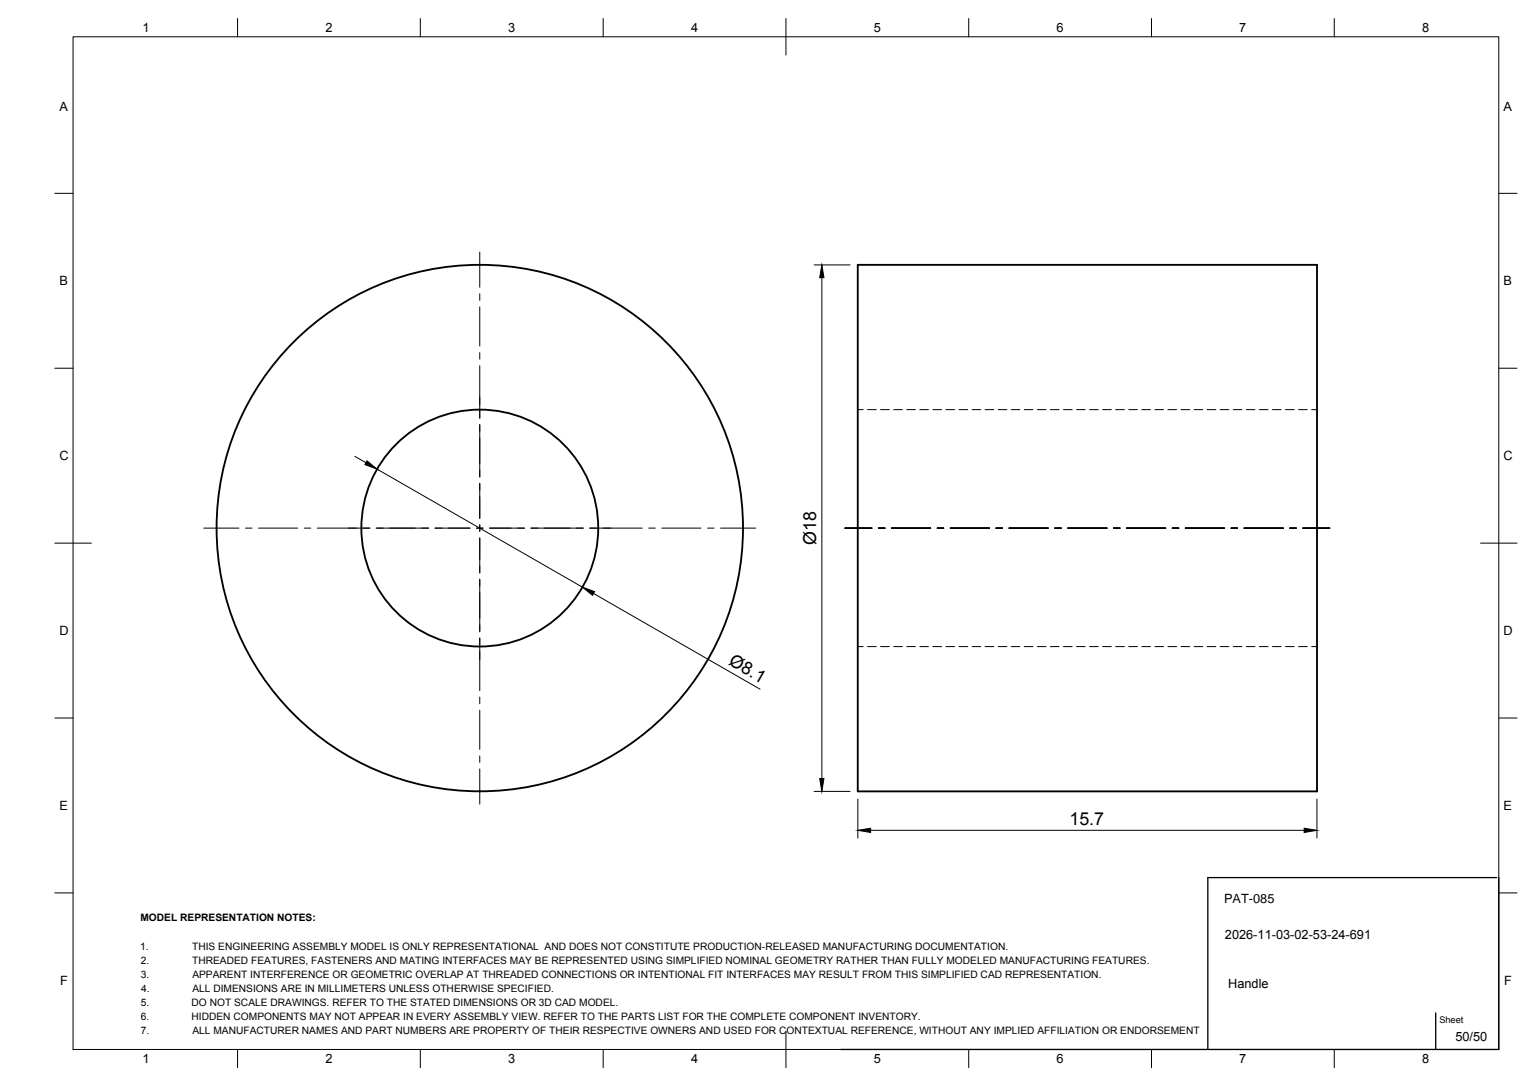
ISO-10303-21;
HEADER;
/* Generated by software containing ST-Developer
 * from STEP Tools, Inc. (www.steptools.com) 
 */

FILE_DESCRIPTION(
/* description */ ('Rack and pinion manual slide'),
/* implementation_level */ '2;1');

FILE_NAME(
/* name */ 'Handle.step',
/* time_stamp */ '2026-10-28T03:22:49-07:00',
/* author */ (''),
/* organization */ (''),
/* preprocessor_version */ 'ST-DEVELOPER v20.2',
/* originating_system */ 'Autodesk Translation Framework v15.17.0.0',
/* authorisation */ '');

FILE_SCHEMA (('AUTOMOTIVE_DESIGN { 1 0 10303 214 3 1 1 }'));
ENDSEC;

DATA;
#10=MECHANICAL_DESIGN_GEOMETRIC_PRESENTATION_REPRESENTATION('',(#784),#34851);
#685=SHAPE_REPRESENTATION_RELATIONSHIP('SRR','None',#35125,#731);
#731=ADVANCED_BREP_SHAPE_REPRESENTATION('',(#832),#34850);
#784=STYLED_ITEM('',(#35404),#832);
#832=MANIFOLD_SOLID_BREP('Body1',#13809);
#1042=FACE_BOUND('',#3221,.T.);
#1043=FACE_BOUND('',#3223,.T.);
#1533=PLANE('',#15593);
#1534=PLANE('',#15594);
#2270=FACE_OUTER_BOUND('',#3218,.T.);
#2271=FACE_OUTER_BOUND('',#3219,.T.);
#2272=FACE_OUTER_BOUND('',#3220,.T.);
#2273=FACE_OUTER_BOUND('',#3222,.T.);
#3218=EDGE_LOOP('',(#12832,#12833,#12834,#12835));
#3219=EDGE_LOOP('',(#12836,#12837,#12838,#12839));
#3220=EDGE_LOOP('',(#12840));
#3221=EDGE_LOOP('',(#12841));
#3222=EDGE_LOOP('',(#12842));
#3223=EDGE_LOOP('',(#12843));
#4513=LINE('',#34729,#5804);
#4514=LINE('',#34735,#5805);
#5804=VECTOR('',#19433,0.404999999999999);
#5805=VECTOR('',#19440,0.9);
#6220=CIRCLE('',#15588,0.404999999999999);
#6221=CIRCLE('',#15589,0.404999999999999);
#6222=CIRCLE('',#15591,0.9);
#6223=CIRCLE('',#15592,0.9);
#7425=VERTEX_POINT('',#34726);
#7426=VERTEX_POINT('',#34728);
#7427=VERTEX_POINT('',#34732);
#7428=VERTEX_POINT('',#34734);
#9228=EDGE_CURVE('',#7425,#7425,#6220,.T.);
#9229=EDGE_CURVE('',#7425,#7426,#4513,.T.);
#9230=EDGE_CURVE('',#7426,#7426,#6221,.T.);
#9231=EDGE_CURVE('',#7427,#7427,#6222,.T.);
#9232=EDGE_CURVE('',#7427,#7428,#4514,.T.);
#9233=EDGE_CURVE('',#7428,#7428,#6223,.T.);
#12832=ORIENTED_EDGE('',*,*,#9228,.F.);
#12833=ORIENTED_EDGE('',*,*,#9229,.T.);
#12834=ORIENTED_EDGE('',*,*,#9230,.T.);
#12835=ORIENTED_EDGE('',*,*,#9229,.F.);
#12836=ORIENTED_EDGE('',*,*,#9231,.F.);
#12837=ORIENTED_EDGE('',*,*,#9232,.T.);
#12838=ORIENTED_EDGE('',*,*,#9233,.T.);
#12839=ORIENTED_EDGE('',*,*,#9232,.F.);
#12840=ORIENTED_EDGE('',*,*,#9231,.T.);
#12841=ORIENTED_EDGE('',*,*,#9228,.T.);
#12842=ORIENTED_EDGE('',*,*,#9233,.F.);
#12843=ORIENTED_EDGE('',*,*,#9230,.F.);
#13011=CYLINDRICAL_SURFACE('',#15587,0.404999999999999);
#13012=CYLINDRICAL_SURFACE('',#15590,0.9);
#13748=ADVANCED_FACE('',(#2270),#13011,.F.);
#13749=ADVANCED_FACE('',(#2271),#13012,.T.);
#13750=ADVANCED_FACE('',(#2272,#1042),#1533,.T.);
#13751=ADVANCED_FACE('',(#2273,#1043),#1534,.F.);
#13809=CLOSED_SHELL('',(#13748,#13749,#13750,#13751));
#15586=AXIS2_PLACEMENT_3D('',#34724,#19427,#19428);
#15587=AXIS2_PLACEMENT_3D('',#34725,#19429,#19430);
#15588=AXIS2_PLACEMENT_3D('',#34727,#19431,#19432);
#15589=AXIS2_PLACEMENT_3D('',#34730,#19434,#19435);
#15590=AXIS2_PLACEMENT_3D('',#34731,#19436,#19437);
#15591=AXIS2_PLACEMENT_3D('',#34733,#19438,#19439);
#15592=AXIS2_PLACEMENT_3D('',#34736,#19441,#19442);
#15593=AXIS2_PLACEMENT_3D('',#34737,#19443,#19444);
#15594=AXIS2_PLACEMENT_3D('',#34738,#19445,#19446);
#19427=DIRECTION('axis',(0.,0.,1.));
#19428=DIRECTION('refdir',(1.,0.,0.));
#19429=DIRECTION('center_axis',(0.,1.,0.));
#19430=DIRECTION('ref_axis',(1.,0.,0.));
#19431=DIRECTION('center_axis',(0.,-1.,0.));
#19432=DIRECTION('ref_axis',(1.,0.,0.));
#19433=DIRECTION('',(0.,-1.,0.));
#19434=DIRECTION('center_axis',(0.,-1.,0.));
#19435=DIRECTION('ref_axis',(1.,0.,0.));
#19436=DIRECTION('center_axis',(0.,1.,0.));
#19437=DIRECTION('ref_axis',(1.,0.,0.));
#19438=DIRECTION('center_axis',(0.,1.,0.));
#19439=DIRECTION('ref_axis',(1.,0.,0.));
#19440=DIRECTION('',(0.,-1.,0.));
#19441=DIRECTION('center_axis',(0.,1.,0.));
#19442=DIRECTION('ref_axis',(1.,0.,0.));
#19443=DIRECTION('center_axis',(0.,1.,0.));
#19444=DIRECTION('ref_axis',(1.,0.,0.));
#19445=DIRECTION('center_axis',(0.,1.,0.));
#19446=DIRECTION('ref_axis',(1.,0.,0.));
#34724=CARTESIAN_POINT('',(0.,0.,0.));
#34725=CARTESIAN_POINT('Origin',(11.,7.3,13.25));
#34726=CARTESIAN_POINT('',(10.595,8.87,13.25));
#34727=CARTESIAN_POINT('Origin',(11.,8.87,13.25));
#34728=CARTESIAN_POINT('',(10.595,7.3,13.25));
#34729=CARTESIAN_POINT('',(10.595,7.3,13.25));
#34730=CARTESIAN_POINT('Origin',(11.,7.3,13.25));
#34731=CARTESIAN_POINT('Origin',(11.,7.3,13.25));
#34732=CARTESIAN_POINT('',(10.1,8.87,13.25));
#34733=CARTESIAN_POINT('Origin',(11.,8.87,13.25));
#34734=CARTESIAN_POINT('',(10.1,7.3,13.25));
#34735=CARTESIAN_POINT('',(10.1,7.3,13.25));
#34736=CARTESIAN_POINT('Origin',(11.,7.3,13.25));
#34737=CARTESIAN_POINT('Origin',(11.,8.87,13.25));
#34738=CARTESIAN_POINT('Origin',(11.,7.3,13.25));
#34796=UNCERTAINTY_MEASURE_WITH_UNIT(LENGTH_MEASURE(0.001),#34852,
'DISTANCE_ACCURACY_VALUE',
'Maximum model space distance between geometric entities at asserted c
onnectivities');
#34797=UNCERTAINTY_MEASURE_WITH_UNIT(LENGTH_MEASURE(0.001),#34852,
'DISTANCE_ACCURACY_VALUE',
'Maximum model space distance between geometric entities at asserted c
onnectivities');
#34850=(
GEOMETRIC_REPRESENTATION_CONTEXT(3)
GLOBAL_UNCERTAINTY_ASSIGNED_CONTEXT((#34796))
GLOBAL_UNIT_ASSIGNED_CONTEXT((#34852,#34854,#34855))
REPRESENTATION_CONTEXT('','3D')
);
#34851=(
GEOMETRIC_REPRESENTATION_CONTEXT(3)
GLOBAL_UNCERTAINTY_ASSIGNED_CONTEXT((#34797))
GLOBAL_UNIT_ASSIGNED_CONTEXT((#34852,#34854,#34855))
REPRESENTATION_CONTEXT('','3D')
);
#34852=(
LENGTH_UNIT()
NAMED_UNIT(*)
SI_UNIT(.CENTI.,.METRE.)
);
#34854=(
NAMED_UNIT(*)
PLANE_ANGLE_UNIT()
SI_UNIT($,.RADIAN.)
);
#34855=(
NAMED_UNIT(*)
SI_UNIT($,.STERADIAN.)
SOLID_ANGLE_UNIT()
);
#34908=SHAPE_DEFINITION_REPRESENTATION(#35067,#35125);
#35067=PRODUCT_DEFINITION_SHAPE('',$,#35179);
#35125=SHAPE_REPRESENTATION('',(#15586),#34850);
#35126=PRODUCT_DEFINITION_CONTEXT('part definition',#35287,'design');
#35179=PRODUCT_DEFINITION('Handle','Handle',#35232,#35126);
#35232=PRODUCT_DEFINITION_FORMATION('',$,#35341);
#35287=APPLICATION_CONTEXT(
'Core Data for Automotive Mechanical Design Process');
#35288=PRODUCT_CONTEXT('part definition',#35287,'mechanical');
#35341=PRODUCT('Handle','Handle','Handle',(#35288));
#35398=COLOUR_RGB('Sky Blue',0.24,0.69,0.87);
#35399=FILL_AREA_STYLE_COLOUR('',#35398);
#35400=FILL_AREA_STYLE('',(#35399));
#35401=SURFACE_STYLE_FILL_AREA(#35400);
#35402=SURFACE_SIDE_STYLE('',(#35401));
#35403=SURFACE_STYLE_USAGE(.BOTH.,#35402);
#35404=PRESENTATION_STYLE_ASSIGNMENT((#35403));
ENDSEC;
END-ISO-10303-21;
